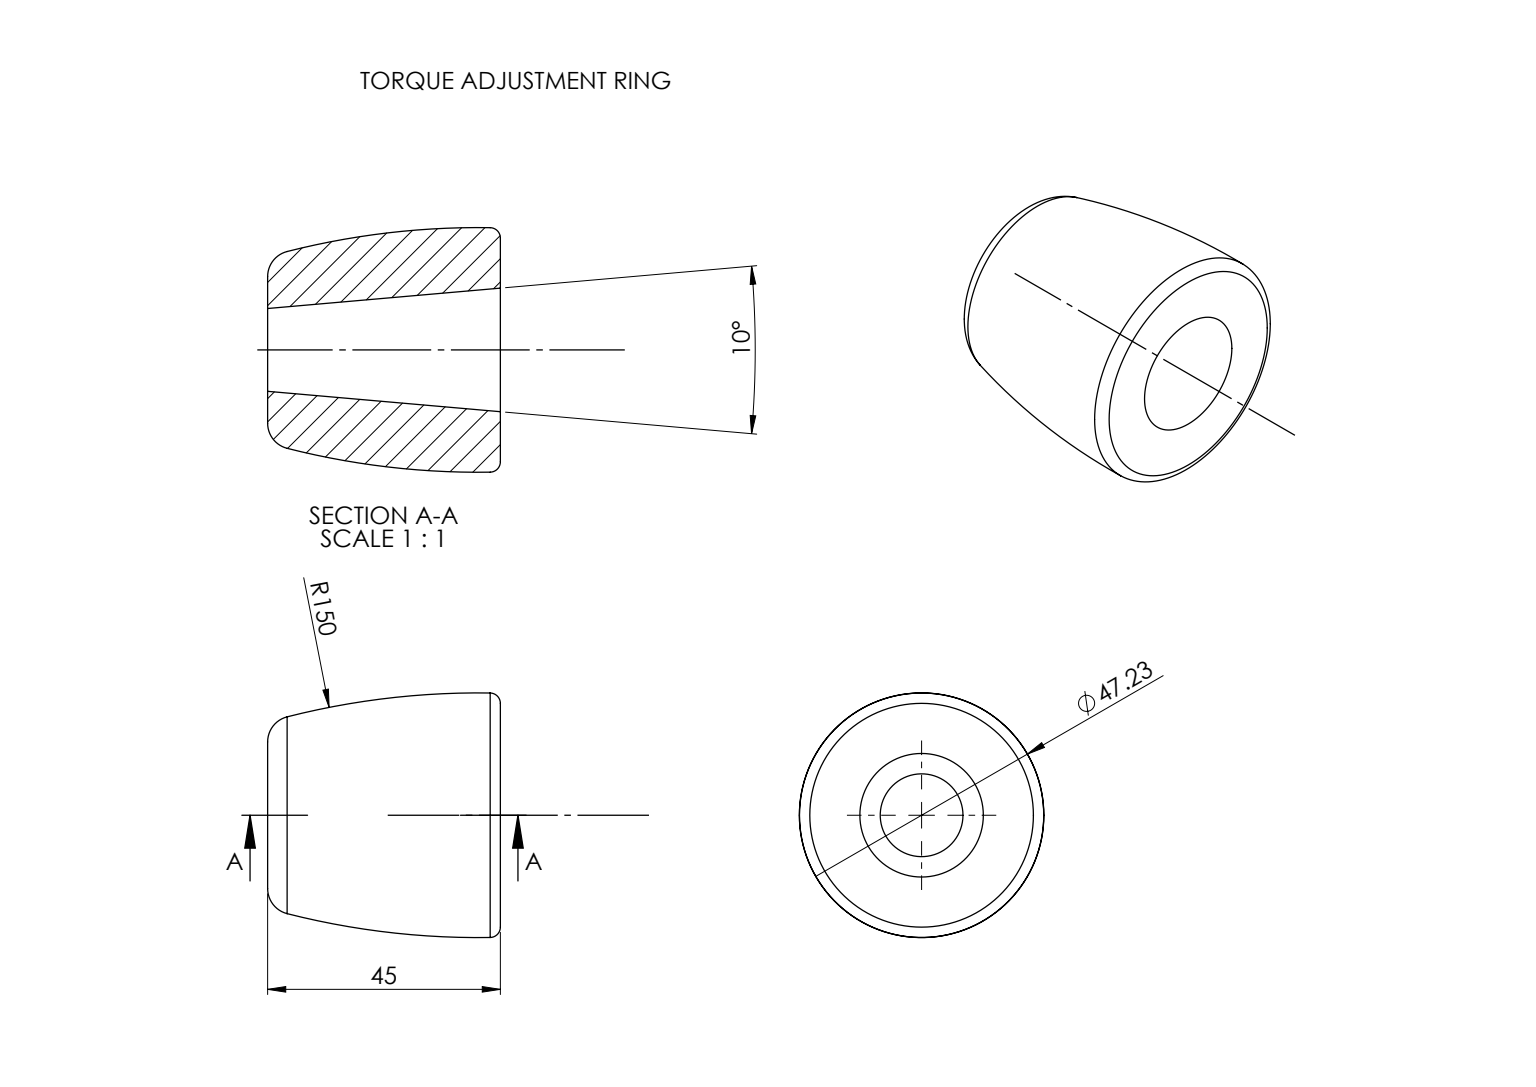
ISO-10303-21;
HEADER;
FILE_DESCRIPTION (('STEP AP214'),
    '1' );
FILE_NAME ('torque adjustment ring.step',
    '2026-10-05T20:22:16',
    ( '' ),
    ( '' ),
    'SwSTEP 2.0',
    'SolidWorks 2026',
    '' );
FILE_SCHEMA (( 'AUTOMOTIVE_DESIGN' ));
ENDSEC;

DATA;
#3=AXIS2_PLACEMENT_3D ( 'NONE', #2045, #12839, #15664 ) ;
#32=CARTESIAN_POINT ( 'NONE',  ( -194.2319660531761656, 171.6227766016838245, -19.01029467089431080 ) ) ;
#233=VERTEX_POINT ( 'NONE', #10201 ) ;
#326=ORIENTED_EDGE ( 'NONE', *, *, #14886, .T. ) ;
#330=DIRECTION ( 'NONE',  ( 0.000000000000000000, 0.000000000000000000, 1.000000000000000000 ) ) ;
#337=EDGE_CURVE ( 'NONE', #3754, #14218, #4437, .T. ) ;
#454=DIRECTION ( 'NONE',  ( 1.000000000000000000, -0.000000000000000000, -0.000000000000000000 ) ) ;
#509=CARTESIAN_POINT ( 'NONE',  ( -192.9999999999999716, 171.6227766016838245, 0.000000000000000000 ) ) ;
#533=CIRCLE ( 'NONE', #811, 21.61734737250326077 ) ;
#595=SURFACE_STYLE_FILL_AREA ( #3338 ) ;
#630=ORIENTED_EDGE ( 'NONE', *, *, #2454, .F. ) ;
#635=UNCERTAINTY_MEASURE_WITH_UNIT (LENGTH_MEASURE( 1.000000000000000082E-05 ), #4493, 'distance_accuracy_value', 'NONE');
#651=ORIENTED_EDGE ( 'NONE', *, *, #1422, .F. ) ;
#765=SHAPE_REPRESENTATION_RELATIONSHIP ( 'NONE' , 'NONE' ,  #5345, #9102 ) ;
#774=CARTESIAN_POINT ( 'NONE',  ( -153.0000000000000284, 171.6227766016838245, 11.93698985866628526 ) ) ;
#802=AXIS2_PLACEMENT_3D ( 'NONE', #9199, #2579, #1331 ) ;
#811=AXIS2_PLACEMENT_3D ( 'NONE', #14678, #15827, #11740 ) ;
#834=AXIS2_PLACEMENT_3D ( 'NONE', #9039, #6477, #17278 ) ;
#856=SURFACE_STYLE_FILL_AREA ( #11204 ) ;
#862=VECTOR ( 'NONE', #2805, 1000.000000000000000 ) ;
#877=CARTESIAN_POINT ( 'NONE',  ( -192.9999999999999716, 171.6227766016838245, 14.16444493696511486 ) ) ;
#976=ORIENTED_EDGE ( 'NONE', *, *, #11728, .F. ) ;
#991=EDGE_CURVE ( 'NONE', #12595, #8470, #13689, .T. ) ;
#1021=DIRECTION ( 'NONE',  ( 0.000000000000000000, 0.000000000000000000, -1.000000000000000000 ) ) ;
#1098=ORIENTED_EDGE ( 'NONE', *, *, #4065, .F. ) ;
#1240=DIRECTION ( 'NONE',  ( 1.000000000000000000, -0.000000000000000000, -0.000000000000000000 ) ) ;
#1247=ORIENTED_EDGE ( 'NONE', *, *, #8739, .F. ) ;
#1259=EDGE_LOOP ( 'NONE', ( #12011, #13058, #12458, #11892 ) ) ;
#1331=DIRECTION ( 'NONE',  ( 0.000000000000000000, 0.000000000000000000, 1.000000000000000000 ) ) ;
#1422=EDGE_CURVE ( 'NONE', #6189, #8470, #2253, .T. ) ;
#1470=CARTESIAN_POINT ( 'NONE',  ( -194.2319660531761656, 171.6227766016838245, 0.000000000000000000 ) ) ;
#1651=PRODUCT_DEFINITION_CONTEXT ( 'detailed design', #14329, 'design' ) ;
#1758=EDGE_CURVE ( 'NONE', #3754, #2297, #9190, .T. ) ;
#1809=DIRECTION ( 'NONE',  ( -1.000000000000000000, 0.000000000000000000, 0.000000000000000000 ) ) ;
#1825=( LENGTH_UNIT ( ) NAMED_UNIT ( * ) SI_UNIT ( .MILLI., .METRE. ) );
#1883=DIRECTION ( 'NONE',  ( 0.000000000000000000, 0.000000000000000000, -1.000000000000000000 ) ) ;
#1930=PRODUCT_DEFINITION_SHAPE ( 'NONE', 'NONE',  #13343 ) ;
#2009=SURFACE_STYLE_USAGE ( .BOTH. , #15288 ) ;
#2045=CARTESIAN_POINT ( 'NONE',  ( -154.9692839938123257, 171.6227766016838245, 0.000000000000000000 ) ) ;
#2150=DIRECTION ( 'NONE',  ( 0.000000000000000000, 0.000000000000000000, -1.000000000000000000 ) ) ;
#2253=CIRCLE ( 'NONE', #4530, 11.93698985866628526 ) ;
#2297=VERTEX_POINT ( 'NONE', #3111 ) ;
#2413=STYLED_ITEM ( 'NONE', ( #10047 ), #5407 ) ;
#2454=EDGE_CURVE ( 'NONE', #14218, #3754, #13004, .T. ) ;
#2479=FACE_OUTER_BOUND ( 'NONE', #7297, .T. ) ;
#2579=DIRECTION ( 'NONE',  ( -1.000000000000000000, 0.000000000000000000, 0.000000000000000000 ) ) ;
#2612=ORIENTED_EDGE ( 'NONE', *, *, #337, .F. ) ;
#2635=ORIENTED_EDGE ( 'NONE', *, *, #4081, .T. ) ;
#2752=DIRECTION ( 'NONE',  ( 0.000000000000000000, 0.000000000000000000, 1.000000000000000000 ) ) ;
#2805=DIRECTION ( 'NONE',  ( 0.9961946980917461003, 1.067350013832217088E-17, 0.08715574274765162943 ) ) ;
#2807=EDGE_LOOP ( 'NONE', ( #651, #12100 ) ) ;
#2978=CARTESIAN_POINT ( 'NONE',  ( -153.0000000000000284, 183.5597664603500903, 0.000000000000000000 ) ) ;
#2979=CARTESIAN_POINT ( 'NONE',  ( -197.9999999999999716, 171.6227766016838245, 0.000000000000000000 ) ) ;
#2986=AXIS2_PLACEMENT_3D ( 'NONE', #2978, #5729, #8206 ) ;
#3008=ORIENTED_EDGE ( 'NONE', *, *, #7683, .F. ) ;
#3045=CARTESIAN_POINT ( 'NONE',  ( -194.2319660531761656, 171.6227766016838245, 19.01029467089431080 ) ) ;
#3111=CARTESIAN_POINT ( 'NONE',  ( -153.0000000000000284, 171.6227766016838245, -21.61734737250326077 ) ) ;
#3112=DIRECTION ( 'NONE',  ( 0.000000000000000000, 0.000000000000000000, -1.000000000000000000 ) ) ;
#3144=PLANE ( 'NONE',  #14534 ) ;
#3163=( LENGTH_UNIT ( ) NAMED_UNIT ( * ) SI_UNIT ( .MILLI., .METRE. ) );
#3172=DIRECTION ( 'NONE',  ( 0.000000000000000000, 0.000000000000000000, -1.000000000000000000 ) ) ;
#3329=ORIENTED_EDGE ( 'NONE', *, *, #991, .F. ) ;
#3338=FILL_AREA_STYLE ('',( #15545 ) ) ;
#3340=DIRECTION ( 'NONE',  ( 0.000000000000000000, 0.000000000000000000, -1.000000000000000000 ) ) ;
#3422=EDGE_CURVE ( 'NONE', #12595, #8077, #4266, .T. ) ;
#3523=DIRECTION ( 'NONE',  ( 0.000000000000000000, -1.000000000000000000, 0.000000000000000000 ) ) ;
#3544=ORIENTED_EDGE ( 'NONE', *, *, #8827, .F. ) ;
#3560=TOROIDAL_SURFACE ( 'NONE', #10616, 21.61734737250326077, 2.000000000000000000 ) ;
#3583=AXIS2_PLACEMENT_3D ( 'NONE', #5482, #6893, #8222 ) ;
#3636=ADVANCED_FACE ( 'NONE', ( #2479 ), #13231, .T. ) ;
#3754=VERTEX_POINT ( 'NONE', #15306 ) ;
#3816=EDGE_LOOP ( 'NONE', ( #16162, #7840, #326, #3008 ) ) ;
#3852=UNCERTAINTY_MEASURE_WITH_UNIT (LENGTH_MEASURE( 1.000000000000000082E-05 ), #3163, 'distance_accuracy_value', 'NONE');
#3928=AXIS2_PLACEMENT_3D ( 'NONE', #13888, #16532, #330 ) ;
#3940=AXIS2_PLACEMENT_3D ( 'NONE', #16610, #11375, #10129 ) ;
#4005=CARTESIAN_POINT ( 'NONE',  ( -197.9999999999999716, 171.6227766016838245, 0.000000000000000000 ) ) ;
#4044=DIRECTION ( 'NONE',  ( 1.000000000000000000, -0.000000000000000000, -0.000000000000000000 ) ) ;
#4065=EDGE_CURVE ( 'NONE', #9320, #13341, #5617, .T. ) ;
#4081=EDGE_CURVE ( 'NONE', #233, #2297, #533, .T. ) ;
#4180=EDGE_CURVE ( 'NONE', #14218, #233, #4215, .T. ) ;
#4215=CIRCLE ( 'NONE', #3928, 2.000000000000001776 ) ;
#4241=ADVANCED_FACE ( 'NONE', ( #6968 ), #5338, .F. ) ;
#4266=CIRCLE ( 'NONE', #16433, 8.000000000000007105 ) ;
#4362=ADVANCED_FACE ( 'NONE', ( #4584 ), #13550, .F. ) ;
#4405=ADVANCED_FACE ( 'NONE', ( #7406 ), #5642, .T. ) ;
#4437=CIRCLE ( 'NONE', #13184, 23.61711149033412127 ) ;
#4493=( LENGTH_UNIT ( ) NAMED_UNIT ( * ) SI_UNIT ( .MILLI., .METRE. ) );
#4495=AXIS2_PLACEMENT_3D ( 'NONE', #2979, #9699, #10855 ) ;
#4514=AXIS2_PLACEMENT_3D ( 'NONE', #8788, #5059, #15676 ) ;
#4530=AXIS2_PLACEMENT_3D ( 'NONE', #12495, #11149, #9829 ) ;
#4574=ORIENTED_EDGE ( 'NONE', *, *, #15169, .T. ) ;
#4584=FACE_OUTER_BOUND ( 'NONE', #16122, .T. ) ;
#4600=EDGE_LOOP ( 'NONE', ( #5693, #2635 ) ) ;
#4704=UNCERTAINTY_MEASURE_WITH_UNIT (LENGTH_MEASURE( 1.000000000000000082E-05 ), #1825, 'distance_accuracy_value', 'NONE');
#4736=CARTESIAN_POINT ( 'NONE',  ( -153.0000000000000284, 171.6227766016838245, 0.000000000000000000 ) ) ;
#4765=PRODUCT ( 'torque adjustment ring', 'torque adjustment ring', '', ( #10225 ) ) ;
#4793=ORIENTED_EDGE ( 'NONE', *, *, #8994, .T. ) ;
#4954=( GEOMETRIC_REPRESENTATION_CONTEXT ( 3 ) GLOBAL_UNCERTAINTY_ASSIGNED_CONTEXT ( ( #3852 ) ) GLOBAL_UNIT_ASSIGNED_CONTEXT ( ( #3163, #14057, #9884 ) ) REPRESENTATION_CONTEXT ( 'NONE', 'WORKASPACE' ) );
#5059=DIRECTION ( 'NONE',  ( -1.000000000000000000, 0.000000000000000000, 0.000000000000000000 ) ) ;
#5113=CIRCLE ( 'NONE', #6533, 21.61734737250326077 ) ;
#5259=CLOSED_SHELL ( 'NONE', ( #11395, #10558, #4241, #14247, #4405, #5362, #4362, #7058, #3636, #8631 ) ) ;
#5338=CONICAL_SURFACE ( 'NONE', #4495, 8.000000000000007105, 0.08726646259970990971 ) ;
#5345=SHAPE_REPRESENTATION ( 'torque adjustment ring', ( #3583 ), #17150 ) ;
#5362=ADVANCED_FACE ( 'NONE', ( #12200, #15098 ), #11118, .T. ) ;
#5407=MANIFOLD_SOLID_BREP ( 'Fillet2', #5259 ) ;
#5482=CARTESIAN_POINT ( 'NONE',  ( 0.000000000000000000, 0.000000000000000000, 0.000000000000000000 ) ) ;
#5529=CARTESIAN_POINT ( 'NONE',  ( -197.9999999999999716, 171.6227766016838245, 0.000000000000000000 ) ) ;
#5617=CIRCLE ( 'NONE', #16375, 5.000000000000000888 ) ;
#5642=TOROIDAL_SURFACE ( 'NONE', #8172, -126.3651973469810628, 149.9999999999999716 ) ;
#5661=ORIENTED_EDGE ( 'NONE', *, *, #15270, .T. ) ;
#5675=ORIENTED_EDGE ( 'NONE', *, *, #4065, .T. ) ;
#5693=ORIENTED_EDGE ( 'NONE', *, *, #8827, .T. ) ;
#5729=DIRECTION ( 'NONE',  ( 1.000000000000000000, 0.000000000000000000, -0.000000000000000000 ) ) ;
#5903=SURFACE_STYLE_USAGE ( .BOTH. , #12624 ) ;
#5996=FILL_AREA_STYLE_COLOUR ( '', #15135 ) ;
#6001=DIRECTION ( 'NONE',  ( 0.000000000000000000, 0.000000000000000000, 1.000000000000000000 ) ) ;
#6048=ORIENTED_EDGE ( 'NONE', *, *, #337, .T. ) ;
#6161=( NAMED_UNIT ( * ) PLANE_ANGLE_UNIT ( ) SI_UNIT ( $, .RADIAN. ) );
#6189=VERTEX_POINT ( 'NONE', #12414 ) ;
#6472=VERTEX_POINT ( 'NONE', #17084 ) ;
#6477=DIRECTION ( 'NONE',  ( -1.000000000000000000, 0.000000000000000000, 0.000000000000000000 ) ) ;
#6533=AXIS2_PLACEMENT_3D ( 'NONE', #4736, #8967, #7464 ) ;
#6570=CARTESIAN_POINT ( 'NONE',  ( -154.9692839938123257, 171.6227766016838245, 0.000000000000000000 ) ) ;
#6696=FACE_OUTER_BOUND ( 'NONE', #11583, .T. ) ;
#6893=DIRECTION ( 'NONE',  ( 0.000000000000000000, 0.000000000000000000, 1.000000000000000000 ) ) ;
#6968=FACE_OUTER_BOUND ( 'NONE', #3816, .T. ) ;
#7035=DIRECTION ( 'NONE',  ( 0.000000000000000000, 0.000000000000000000, -1.000000000000000000 ) ) ;
#7042=CIRCLE ( 'NONE', #3940, 11.93698985866628526 ) ;
#7058=ADVANCED_FACE ( 'NONE', ( #16779, #10211 ), #3144, .T. ) ;
#7157=ORIENTED_EDGE ( 'NONE', *, *, #9878, .F. ) ;
#7228=AXIS2_PLACEMENT_3D ( 'NONE', #16086, #15812, #1021 ) ;
#7229=CARTESIAN_POINT ( 'NONE',  ( -197.9999999999999716, 171.6227766016838245, 0.000000000000000000 ) ) ;
#7262=VERTEX_POINT ( 'NONE', #32 ) ;
#7268=DIRECTION ( 'NONE',  ( -0.000000000000000000, -1.000000000000000000, -0.000000000000000000 ) ) ;
#7273=CIRCLE ( 'NONE', #13781, 8.000000000000007105 ) ;
#7297=EDGE_LOOP ( 'NONE', ( #7157, #14624, #5675, #9515 ) ) ;
#7341=CIRCLE ( 'NONE', #4514, 14.16444493696511486 ) ;
#7406=FACE_OUTER_BOUND ( 'NONE', #11127, .T. ) ;
#7464=DIRECTION ( 'NONE',  ( 0.000000000000000000, 0.000000000000000000, -1.000000000000000000 ) ) ;
#7683=EDGE_CURVE ( 'NONE', #8077, #6189, #12298, .T. ) ;
#7746=ORIENTED_EDGE ( 'NONE', *, *, #7683, .T. ) ;
#7837=PRODUCT_DEFINITION_FORMATION_WITH_SPECIFIED_SOURCE ( 'ANY', '', #4765, .NOT_KNOWN. ) ;
#7840=ORIENTED_EDGE ( 'NONE', *, *, #991, .T. ) ;
#7944=AXIS2_PLACEMENT_3D ( 'NONE', #1470, #4044, #9506 ) ;
#7980=DIRECTION ( 'NONE',  ( -1.000000000000000000, 0.000000000000000000, 0.000000000000000000 ) ) ;
#8077=VERTEX_POINT ( 'NONE', #10598 ) ;
#8172=AXIS2_PLACEMENT_3D ( 'NONE', #12808, #16880, #11301 ) ;
#8206=DIRECTION ( 'NONE',  ( -0.000000000000000000, 0.000000000000000000, -1.000000000000000000 ) ) ;
#8215=FACE_OUTER_BOUND ( 'NONE', #12687, .T. ) ;
#8222=DIRECTION ( 'NONE',  ( 1.000000000000000000, 0.000000000000000000, 0.000000000000000000 ) ) ;
#8277=CARTESIAN_POINT ( 'NONE',  ( -157.2729844578908001, 171.6227766016837961, -126.3651973469810628 ) ) ;
#8396=STYLED_ITEM ( 'NONE', ( #12723 ), #9102 ) ;
#8470=VERTEX_POINT ( 'NONE', #774 ) ;
#8511=CARTESIAN_POINT ( 'NONE',  ( -157.2729844578908001, 171.6227766016838245, 126.3651973469810628 ) ) ;
#8631=ADVANCED_FACE ( 'NONE', ( #6696 ), #14724, .T. ) ;
#8739=EDGE_CURVE ( 'NONE', #7262, #9320, #14175, .T. ) ;
#8788=CARTESIAN_POINT ( 'NONE',  ( -197.9999999999999716, 171.6227766016838245, 0.000000000000000000 ) ) ;
#8827=EDGE_CURVE ( 'NONE', #2297, #233, #5113, .T. ) ;
#8892=DIRECTION ( 'NONE',  ( 1.000000000000000000, -0.000000000000000000, -0.000000000000000000 ) ) ;
#8911=DIRECTION ( 'NONE',  ( 0.000000000000000000, 0.000000000000000000, -1.000000000000000000 ) ) ;
#8927=ORIENTED_EDGE ( 'NONE', *, *, #4180, .T. ) ;
#8958=EDGE_CURVE ( 'NONE', #7262, #3754, #9358, .T. ) ;
#8967=DIRECTION ( 'NONE',  ( 1.000000000000000000, -0.000000000000000000, -0.000000000000000000 ) ) ;
#8994=EDGE_CURVE ( 'NONE', #9320, #7262, #11891, .T. ) ;
#9039=CARTESIAN_POINT ( 'NONE',  ( -197.9999999999999716, 171.6227766016838245, 0.000000000000000000 ) ) ;
#9102=ADVANCED_BREP_SHAPE_REPRESENTATION ( '', ( #5407, #3583 ), #17150 ) ;
#9190=CIRCLE ( 'NONE', #7228, 2.000000000000001776 ) ;
#9199=CARTESIAN_POINT ( 'NONE',  ( -192.9999999999999716, 171.6227766016838245, 0.000000000000000000 ) ) ;
#9320=VERTEX_POINT ( 'NONE', #3045 ) ;
#9358=CIRCLE ( 'NONE', #10478, 149.9999999999999716 ) ;
#9506=DIRECTION ( 'NONE',  ( 0.000000000000000000, 0.000000000000000000, -1.000000000000000000 ) ) ;
#9515=ORIENTED_EDGE ( 'NONE', *, *, #15169, .F. ) ;
#9601=ORIENTED_EDGE ( 'NONE', *, *, #15270, .F. ) ;
#9675=SHAPE_DEFINITION_REPRESENTATION ( #1930, #5345 ) ;
#9699=DIRECTION ( 'NONE',  ( 1.000000000000000000, -0.000000000000000000, -0.000000000000000000 ) ) ;
#9760=ORIENTED_EDGE ( 'NONE', *, *, #1758, .F. ) ;
#9829=DIRECTION ( 'NONE',  ( 0.000000000000000000, 0.000000000000000000, -1.000000000000000000 ) ) ;
#9878=EDGE_CURVE ( 'NONE', #7262, #6472, #12697, .T. ) ;
#9884=( NAMED_UNIT ( * ) SI_UNIT ( $, .STERADIAN. ) SOLID_ANGLE_UNIT ( ) );
#10006=CARTESIAN_POINT ( 'NONE',  ( -154.9692839938123257, 171.6227766016838245, 23.61711149033413903 ) ) ;
#10026=CARTESIAN_POINT ( 'NONE',  ( -197.9999999999999716, 189.6227766016838245, 0.000000000000000000 ) ) ;
#10047=PRESENTATION_STYLE_ASSIGNMENT (( #2009 ) ) ;
#10129=DIRECTION ( 'NONE',  ( 0.000000000000000000, 0.000000000000000000, -1.000000000000000000 ) ) ;
#10201=CARTESIAN_POINT ( 'NONE',  ( -153.0000000000000284, 171.6227766016838245, 21.61734737250326077 ) ) ;
#10211=FACE_BOUND ( 'NONE', #14710, .T. ) ;
#10225=PRODUCT_CONTEXT ( 'NONE', #13664, 'mechanical' ) ;
#10478=AXIS2_PLACEMENT_3D ( 'NONE', #8511, #7268, #3112 ) ;
#10558=ADVANCED_FACE ( 'NONE', ( #16799 ), #13848, .T. ) ;
#10598=CARTESIAN_POINT ( 'NONE',  ( -197.9999999999999716, 171.6227766016838245, -8.000000000000007105 ) ) ;
#10616=AXIS2_PLACEMENT_3D ( 'NONE', #15106, #15297, #3172 ) ;
#10714=AXIS2_PLACEMENT_3D ( 'NONE', #7229, #8892, #3340 ) ;
#10718=CARTESIAN_POINT ( 'NONE',  ( -192.9999999999999716, 171.6227766016838245, -14.16444493696511486 ) ) ;
#10725=AXIS2_PLACEMENT_3D ( 'NONE', #509, #12812, #6001 ) ;
#10727=CIRCLE ( 'NONE', #834, 14.16444493696511486 ) ;
#10767=CARTESIAN_POINT ( 'NONE',  ( -155.0000000000000284, 171.6227766016838245, 0.000000000000000000 ) ) ;
#10796=ORIENTED_EDGE ( 'NONE', *, *, #1422, .T. ) ;
#10855=DIRECTION ( 'NONE',  ( 0.000000000000000000, 0.000000000000000000, -1.000000000000000000 ) ) ;
#11014=DIRECTION ( 'NONE',  ( 1.000000000000000000, -0.000000000000000000, -0.000000000000000000 ) ) ;
#11022=DIRECTION ( 'NONE',  ( 0.000000000000000000, 0.000000000000000000, -1.000000000000000000 ) ) ;
#11032=CARTESIAN_POINT ( 'NONE',  ( -197.9999999999999716, 171.6227766016838245, 8.000000000000007105 ) ) ;
#11062=CARTESIAN_POINT ( 'NONE',  ( -197.9999999999999716, 171.6227766016838245, -8.000000000000007105 ) ) ;
#11118=PLANE ( 'NONE',  #2986 ) ;
#11127=EDGE_LOOP ( 'NONE', ( #976, #4793, #13727, #6048 ) ) ;
#11149=DIRECTION ( 'NONE',  ( 1.000000000000000000, -0.000000000000000000, -0.000000000000000000 ) ) ;
#11172=ORIENTED_EDGE ( 'NONE', *, *, #9878, .T. ) ;
#11192=DIRECTION ( 'NONE',  ( 0.000000000000000000, 1.000000000000000000, -1.224646799147353207E-16 ) ) ;
#11204=FILL_AREA_STYLE ('',( #5996 ) ) ;
#11301=DIRECTION ( 'NONE',  ( 0.000000000000000000, 0.000000000000000000, -1.000000000000000000 ) ) ;
#11352=FACE_OUTER_BOUND ( 'NONE', #1259, .T. ) ;
#11373=DIRECTION ( 'NONE',  ( 1.000000000000000000, -0.000000000000000000, -0.000000000000000000 ) ) ;
#11375=DIRECTION ( 'NONE',  ( 1.000000000000000000, -0.000000000000000000, -0.000000000000000000 ) ) ;
#11384=( NAMED_UNIT ( * ) SI_UNIT ( $, .STERADIAN. ) SOLID_ANGLE_UNIT ( ) );
#11395=ADVANCED_FACE ( 'NONE', ( #8215 ), #3560, .T. ) ;
#11583=EDGE_LOOP ( 'NONE', ( #15942, #2612, #16217, #16107 ) ) ;
#11624=DIRECTION ( 'NONE',  ( 0.000000000000000000, 0.000000000000000000, 1.000000000000000000 ) ) ;
#11728=EDGE_CURVE ( 'NONE', #9320, #14218, #14298, .T. ) ;
#11740=DIRECTION ( 'NONE',  ( 0.000000000000000000, 0.000000000000000000, -1.000000000000000000 ) ) ;
#11891=CIRCLE ( 'NONE', #7944, 19.01029467089431080 ) ;
#11892=ORIENTED_EDGE ( 'NONE', *, *, #8958, .F. ) ;
#12011=ORIENTED_EDGE ( 'NONE', *, *, #8739, .T. ) ;
#12088=ORIENTED_EDGE ( 'NONE', *, *, #12828, .F. ) ;
#12100=ORIENTED_EDGE ( 'NONE', *, *, #14886, .F. ) ;
#12200=FACE_OUTER_BOUND ( 'NONE', #4600, .T. ) ;
#12298=LINE ( 'NONE', #11062, #15828 ) ;
#12353=CARTESIAN_POINT ( 'NONE',  ( -194.2319660531761656, 171.6227766016838245, 0.000000000000000000 ) ) ;
#12414=CARTESIAN_POINT ( 'NONE',  ( -153.0000000000000284, 171.6227766016838245, -11.93698985866628526 ) ) ;
#12458=ORIENTED_EDGE ( 'NONE', *, *, #2454, .T. ) ;
#12495=CARTESIAN_POINT ( 'NONE',  ( -153.0000000000000284, 171.6227766016838245, 0.000000000000000000 ) ) ;
#12595=VERTEX_POINT ( 'NONE', #15712 ) ;
#12624=SURFACE_SIDE_STYLE ('',( #595 ) ) ;
#12639=( GEOMETRIC_REPRESENTATION_CONTEXT ( 3 ) GLOBAL_UNCERTAINTY_ASSIGNED_CONTEXT ( ( #4704 ) ) GLOBAL_UNIT_ASSIGNED_CONTEXT ( ( #1825, #14055, #11384 ) ) REPRESENTATION_CONTEXT ( 'NONE', 'WORKASPACE' ) );
#12645=EDGE_LOOP ( 'NONE', ( #5661, #4574 ) ) ;
#12687=EDGE_LOOP ( 'NONE', ( #630, #8927, #3544, #9760 ) ) ;
#12697=CIRCLE ( 'NONE', #13546, 5.000000000000000888 ) ;
#12723=PRESENTATION_STYLE_ASSIGNMENT (( #5903 ) ) ;
#12772=CARTESIAN_POINT ( 'NONE',  ( -157.2729844578908001, 171.6227766016838245, 0.000000000000000000 ) ) ;
#12798=ORIENTED_EDGE ( 'NONE', *, *, #12828, .T. ) ;
#12808=CARTESIAN_POINT ( 'NONE',  ( -157.2729844578908001, 171.6227766016838245, 0.000000000000000000 ) ) ;
#12812=DIRECTION ( 'NONE',  ( -1.000000000000000000, 0.000000000000000000, 0.000000000000000000 ) ) ;
#12828=EDGE_CURVE ( 'NONE', #8077, #12595, #7273, .T. ) ;
#12839=DIRECTION ( 'NONE',  ( -1.000000000000000000, 0.000000000000000000, 0.000000000000000000 ) ) ;
#12885=( NAMED_UNIT ( * ) SI_UNIT ( $, .STERADIAN. ) SOLID_ANGLE_UNIT ( ) );
#12963=AXIS2_PLACEMENT_3D ( 'NONE', #12772, #454, #1883 ) ;
#13004=CIRCLE ( 'NONE', #3, 23.61711149033412127 ) ;
#13058=ORIENTED_EDGE ( 'NONE', *, *, #11728, .T. ) ;
#13184=AXIS2_PLACEMENT_3D ( 'NONE', #6570, #7980, #17362 ) ;
#13231=TOROIDAL_SURFACE ( 'NONE', #802, 14.16444493696511486, 5.000000000000000000 ) ;
#13341=VERTEX_POINT ( 'NONE', #14681 ) ;
#13343=PRODUCT_DEFINITION ( 'UNKNOWN', '', #7837, #1651 ) ;
#13546=AXIS2_PLACEMENT_3D ( 'NONE', #10718, #14787, #2752 ) ;
#13550=CONICAL_SURFACE ( 'NONE', #10714, 8.000000000000007105, 0.08726646259970990971 ) ;
#13664=APPLICATION_CONTEXT ( 'automotive_design' ) ;
#13686=DIRECTION ( 'NONE',  ( 0.000000000000000000, 1.850371707708594563E-16, 1.000000000000000000 ) ) ;
#13689=LINE ( 'NONE', #11032, #862 ) ;
#13727=ORIENTED_EDGE ( 'NONE', *, *, #8958, .T. ) ;
#13781=AXIS2_PLACEMENT_3D ( 'NONE', #4005, #1240, #2150 ) ;
#13848=TOROIDAL_SURFACE ( 'NONE', #10725, 14.16444493696511486, 5.000000000000000000 ) ;
#13888=CARTESIAN_POINT ( 'NONE',  ( -155.0000000000000284, 171.6227766016838245, 21.61734737250326077 ) ) ;
#14055=( NAMED_UNIT ( * ) PLANE_ANGLE_UNIT ( ) SI_UNIT ( $, .RADIAN. ) );
#14057=( NAMED_UNIT ( * ) PLANE_ANGLE_UNIT ( ) SI_UNIT ( $, .RADIAN. ) );
#14175=CIRCLE ( 'NONE', #15005, 19.01029467089431080 ) ;
#14218=VERTEX_POINT ( 'NONE', #10006 ) ;
#14247=ADVANCED_FACE ( 'NONE', ( #11352 ), #14378, .T. ) ;
#14293=EDGE_LOOP ( 'NONE', ( #1247, #11172, #9601, #1098 ) ) ;
#14298=CIRCLE ( 'NONE', #16279, 149.9999999999999716 ) ;
#14329=APPLICATION_CONTEXT ( 'automotive_design' ) ;
#14338=COLOUR_RGB ( '', 0.66274510, 0.83137255, 0.94901961) ;
#14378=TOROIDAL_SURFACE ( 'NONE', #12963, -126.3651973469810628, 149.9999999999999716 ) ;
#14534=AXIS2_PLACEMENT_3D ( 'NONE', #10026, #1809, #11624 ) ;
#14624=ORIENTED_EDGE ( 'NONE', *, *, #8994, .F. ) ;
#14678=CARTESIAN_POINT ( 'NONE',  ( -153.0000000000000284, 171.6227766016838245, 0.000000000000000000 ) ) ;
#14681=CARTESIAN_POINT ( 'NONE',  ( -197.9999999999999716, 171.6227766016838245, 14.16444493696511486 ) ) ;
#14710=EDGE_LOOP ( 'NONE', ( #12798, #17162 ) ) ;
#14713=AXIS2_PLACEMENT_3D ( 'NONE', #10767, #16178, #15353 ) ;
#14724=TOROIDAL_SURFACE ( 'NONE', #14713, 21.61734737250326077, 2.000000000000000000 ) ;
#14787=DIRECTION ( 'NONE',  ( 0.000000000000000000, 1.000000000000000000, 1.224646799147353207E-16 ) ) ;
#14886=EDGE_CURVE ( 'NONE', #8470, #6189, #7042, .T. ) ;
#15005=AXIS2_PLACEMENT_3D ( 'NONE', #12353, #11373, #11022 ) ;
#15040=DIRECTION ( 'NONE',  ( 0.9961946980917461003, 0.000000000000000000, -0.08715574274765162943 ) ) ;
#15098=FACE_BOUND ( 'NONE', #2807, .T. ) ;
#15106=CARTESIAN_POINT ( 'NONE',  ( -155.0000000000000284, 171.6227766016838245, 0.000000000000000000 ) ) ;
#15135=COLOUR_RGB ( '', 0.66274510, 0.83137255, 0.94901961) ;
#15169=EDGE_CURVE ( 'NONE', #6472, #13341, #10727, .T. ) ;
#15270=EDGE_CURVE ( 'NONE', #13341, #6472, #7341, .T. ) ;
#15288=SURFACE_SIDE_STYLE ('',( #856 ) ) ;
#15297=DIRECTION ( 'NONE',  ( 1.000000000000000000, -0.000000000000000000, -0.000000000000000000 ) ) ;
#15306=CARTESIAN_POINT ( 'NONE',  ( -154.9692839938123257, 171.6227766016838245, -23.61711149033413903 ) ) ;
#15353=DIRECTION ( 'NONE',  ( 0.000000000000000000, 0.000000000000000000, -1.000000000000000000 ) ) ;
#15545=FILL_AREA_STYLE_COLOUR ( '', #14338 ) ;
#15664=DIRECTION ( 'NONE',  ( 0.000000000000000000, 0.000000000000000000, 1.000000000000000000 ) ) ;
#15676=DIRECTION ( 'NONE',  ( 0.000000000000000000, 0.000000000000000000, 1.000000000000000000 ) ) ;
#15712=CARTESIAN_POINT ( 'NONE',  ( -197.9999999999999716, 171.6227766016838245, 8.000000000000007105 ) ) ;
#15751=MECHANICAL_DESIGN_GEOMETRIC_PRESENTATION_REPRESENTATION('',(#8396),#12639);
#15812=DIRECTION ( 'NONE',  ( -0.000000000000000000, -1.000000000000000000, -0.000000000000000000 ) ) ;
#15827=DIRECTION ( 'NONE',  ( 1.000000000000000000, -0.000000000000000000, -0.000000000000000000 ) ) ;
#15828=VECTOR ( 'NONE', #15040, 1000.000000000000000 ) ;
#15942=ORIENTED_EDGE ( 'NONE', *, *, #4180, .F. ) ;
#16086=CARTESIAN_POINT ( 'NONE',  ( -155.0000000000000284, 171.6227766016838245, -21.61734737250326077 ) ) ;
#16107=ORIENTED_EDGE ( 'NONE', *, *, #4081, .F. ) ;
#16122=EDGE_LOOP ( 'NONE', ( #3329, #12088, #7746, #10796 ) ) ;
#16162=ORIENTED_EDGE ( 'NONE', *, *, #3422, .F. ) ;
#16178=DIRECTION ( 'NONE',  ( 1.000000000000000000, -0.000000000000000000, -0.000000000000000000 ) ) ;
#16217=ORIENTED_EDGE ( 'NONE', *, *, #1758, .T. ) ;
#16278=MECHANICAL_DESIGN_GEOMETRIC_PRESENTATION_REPRESENTATION('',(#2413),#4954);
#16279=AXIS2_PLACEMENT_3D ( 'NONE', #8277, #11192, #13686 ) ;
#16375=AXIS2_PLACEMENT_3D ( 'NONE', #877, #3523, #8911 ) ;
#16433=AXIS2_PLACEMENT_3D ( 'NONE', #5529, #11014, #7035 ) ;
#16532=DIRECTION ( 'NONE',  ( 0.000000000000000000, 1.000000000000000000, -1.224646799147353207E-16 ) ) ;
#16610=CARTESIAN_POINT ( 'NONE',  ( -153.0000000000000284, 171.6227766016838245, 0.000000000000000000 ) ) ;
#16779=FACE_OUTER_BOUND ( 'NONE', #12645, .T. ) ;
#16799=FACE_OUTER_BOUND ( 'NONE', #14293, .T. ) ;
#16880=DIRECTION ( 'NONE',  ( 1.000000000000000000, -0.000000000000000000, -0.000000000000000000 ) ) ;
#17084=CARTESIAN_POINT ( 'NONE',  ( -197.9999999999999716, 171.6227766016838245, -14.16444493696511486 ) ) ;
#17150=( GEOMETRIC_REPRESENTATION_CONTEXT ( 3 ) GLOBAL_UNCERTAINTY_ASSIGNED_CONTEXT ( ( #635 ) ) GLOBAL_UNIT_ASSIGNED_CONTEXT ( ( #4493, #6161, #12885 ) ) REPRESENTATION_CONTEXT ( 'NONE', 'WORKASPACE' ) );
#17162=ORIENTED_EDGE ( 'NONE', *, *, #3422, .T. ) ;
#17278=DIRECTION ( 'NONE',  ( 0.000000000000000000, 0.000000000000000000, 1.000000000000000000 ) ) ;
#17362=DIRECTION ( 'NONE',  ( 0.000000000000000000, 0.000000000000000000, 1.000000000000000000 ) ) ;
ENDSEC;
END-ISO-10303-21;
